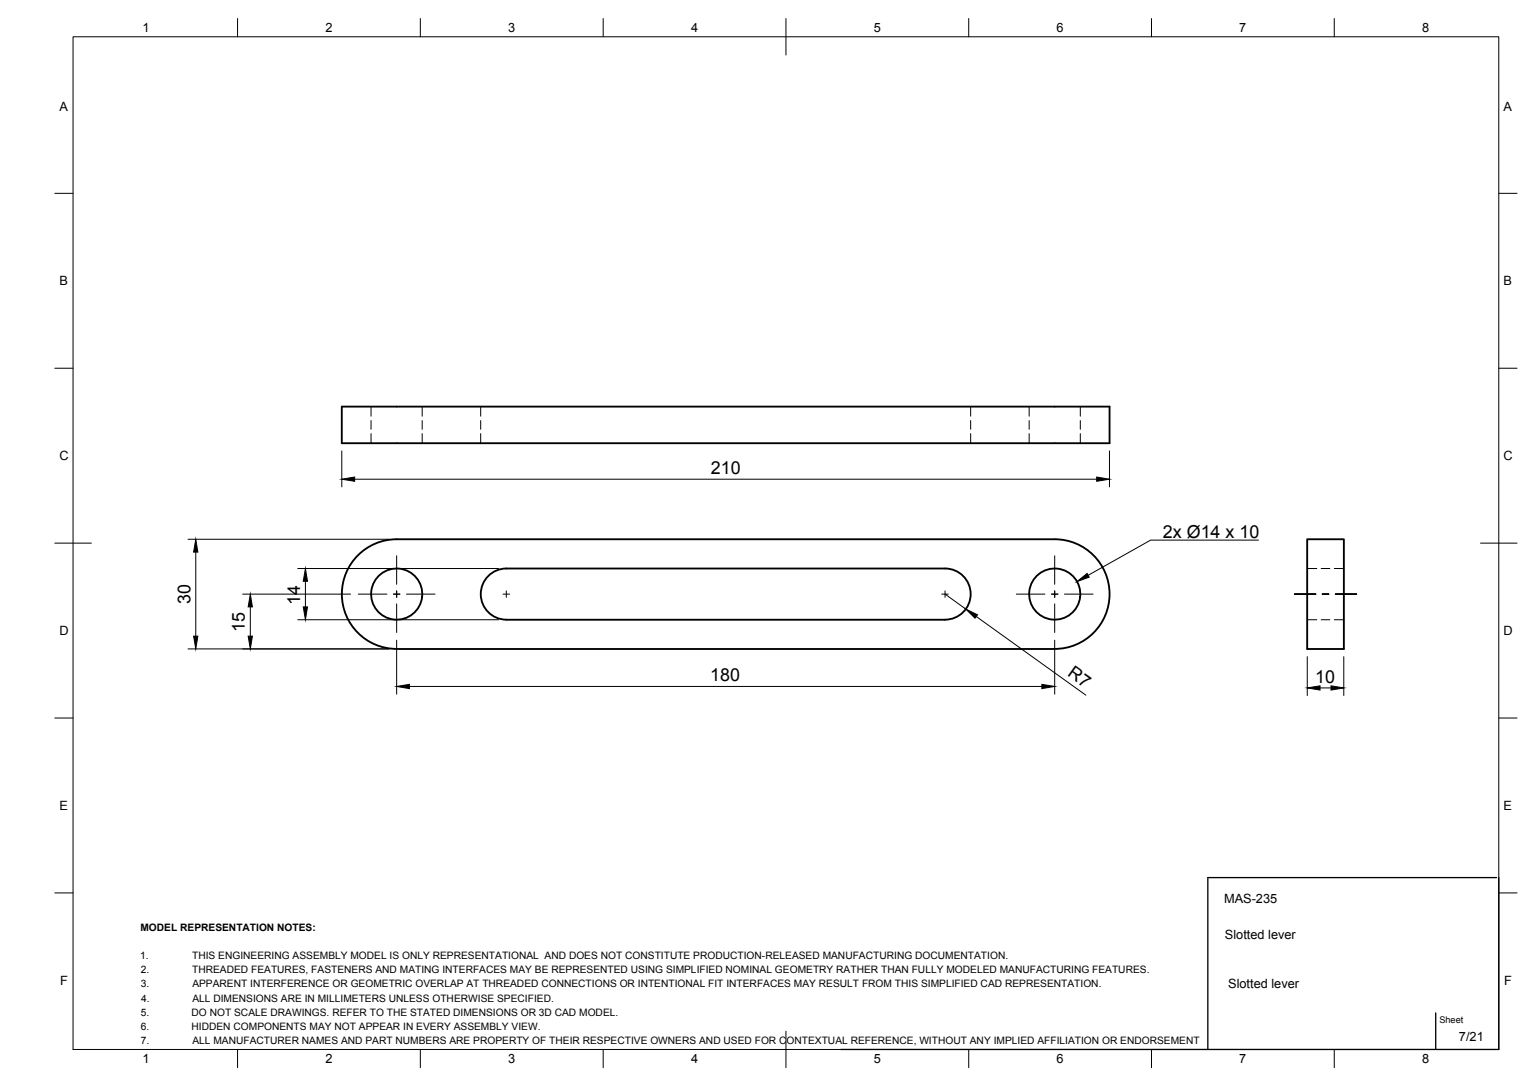
ISO-10303-21;
HEADER;
/* Generated by software containing ST-Developer
 * from STEP Tools, Inc. (www.steptools.com) 
 */

FILE_DESCRIPTION(
/* description */ ('Independent Whitworth quick-return mechanism. Crank radius40, ground-
center spacing80, lever180, connecting rod160, output guide X200. Nomi
nal stroke180 and long/short phase ratio2. Retained guide rods, replac
eable bearing sleeves and captured sliding shoe. No load or production
 rating assigned.'),
/* implementation_level */ '2;1');

FILE_NAME(
/* name */ 'Slotted lever.step',
/* time_stamp */ '2026-11-09T18:22:56-08:00',
/* author */ (''),
/* organization */ (''),
/* preprocessor_version */ 'ST-DEVELOPER v20.2',
/* originating_system */ 'Autodesk Translation Framework v15.17.0.0',
/* authorisation */ '');

FILE_SCHEMA (('AUTOMOTIVE_DESIGN { 1 0 10303 214 3 1 1 }'));
ENDSEC;

DATA;
#10=MECHANICAL_DESIGN_GEOMETRIC_PRESENTATION_REPRESENTATION('',(#223),#4388);
#183=SHAPE_REPRESENTATION_RELATIONSHIP('SRR','None',#4482,#203);
#203=ADVANCED_BREP_SHAPE_REPRESENTATION('',(#243),#4372);
#223=STYLED_ITEM('',(#4590),#243);
#243=MANIFOLD_SOLID_BREP('Body1',#2328);
#271=FACE_BOUND('',#599,.T.);
#272=FACE_BOUND('',#600,.T.);
#273=FACE_BOUND('',#601,.T.);
#274=FACE_BOUND('',#603,.T.);
#275=FACE_BOUND('',#604,.T.);
#276=FACE_BOUND('',#605,.T.);
#333=PLANE('',#2615);
#334=PLANE('',#2619);
#335=PLANE('',#2629);
#336=PLANE('',#2633);
#337=PLANE('',#2637);
#338=PLANE('',#2638);
#429=FACE_OUTER_BOUND('',#588,.T.);
#430=FACE_OUTER_BOUND('',#589,.T.);
#431=FACE_OUTER_BOUND('',#590,.T.);
#432=FACE_OUTER_BOUND('',#591,.T.);
#433=FACE_OUTER_BOUND('',#592,.T.);
#434=FACE_OUTER_BOUND('',#593,.T.);
#435=FACE_OUTER_BOUND('',#594,.T.);
#436=FACE_OUTER_BOUND('',#595,.T.);
#437=FACE_OUTER_BOUND('',#596,.T.);
#438=FACE_OUTER_BOUND('',#597,.T.);
#439=FACE_OUTER_BOUND('',#598,.T.);
#440=FACE_OUTER_BOUND('',#602,.T.);
#588=EDGE_LOOP('',(#1690,#1691,#1692,#1693));
#589=EDGE_LOOP('',(#1694,#1695,#1696,#1697));
#590=EDGE_LOOP('',(#1698,#1699,#1700,#1701));
#591=EDGE_LOOP('',(#1702,#1703,#1704,#1705));
#592=EDGE_LOOP('',(#1706,#1707,#1708,#1709));
#593=EDGE_LOOP('',(#1710,#1711,#1712,#1713));
#594=EDGE_LOOP('',(#1714,#1715,#1716,#1717));
#595=EDGE_LOOP('',(#1718,#1719,#1720,#1721));
#596=EDGE_LOOP('',(#1722,#1723,#1724,#1725));
#597=EDGE_LOOP('',(#1726,#1727,#1728,#1729));
#598=EDGE_LOOP('',(#1730,#1731,#1732,#1733));
#599=EDGE_LOOP('',(#1734,#1735,#1736,#1737));
#600=EDGE_LOOP('',(#1738));
#601=EDGE_LOOP('',(#1739));
#602=EDGE_LOOP('',(#1740,#1741,#1742,#1743));
#603=EDGE_LOOP('',(#1744,#1745,#1746,#1747));
#604=EDGE_LOOP('',(#1748));
#605=EDGE_LOOP('',(#1749));
#787=LINE('',#3813,#926);
#788=LINE('',#3815,#927);
#789=LINE('',#3817,#928);
#790=LINE('',#3818,#929);
#791=LINE('',#3823,#930);
#792=LINE('',#3827,#931);
#793=LINE('',#3829,#932);
#794=LINE('',#3830,#933);
#795=LINE('',#3838,#934);
#796=LINE('',#3844,#935);
#797=LINE('',#3849,#936);
#798=LINE('',#3851,#937);
#799=LINE('',#3853,#938);
#800=LINE('',#3854,#939);
#801=LINE('',#3860,#940);
#802=LINE('',#3863,#941);
#803=LINE('',#3865,#942);
#804=LINE('',#3866,#943);
#926=VECTOR('',#3027,10.);
#927=VECTOR('',#3028,10.);
#928=VECTOR('',#3029,10.);
#929=VECTOR('',#3030,10.);
#930=VECTOR('',#3035,10.);
#931=VECTOR('',#3040,10.);
#932=VECTOR('',#3041,10.);
#933=VECTOR('',#3042,10.);
#934=VECTOR('',#3053,7.);
#935=VECTOR('',#3060,7.);
#936=VECTOR('',#3065,10.);
#937=VECTOR('',#3066,10.);
#938=VECTOR('',#3067,10.);
#939=VECTOR('',#3068,10.);
#940=VECTOR('',#3075,10.);
#941=VECTOR('',#3078,10.);
#942=VECTOR('',#3079,10.);
#943=VECTOR('',#3080,10.);
#1057=CIRCLE('',#2617,7.);
#1058=CIRCLE('',#2618,7.);
#1059=CIRCLE('',#2621,7.);
#1060=CIRCLE('',#2622,7.);
#1061=CIRCLE('',#2624,7.);
#1062=CIRCLE('',#2625,7.);
#1063=CIRCLE('',#2627,7.);
#1064=CIRCLE('',#2628,7.);
#1065=CIRCLE('',#2631,15.);
#1066=CIRCLE('',#2632,15.);
#1067=CIRCLE('',#2635,15.);
#1068=CIRCLE('',#2636,15.);
#1191=VERTEX_POINT('',#3811);
#1192=VERTEX_POINT('',#3812);
#1193=VERTEX_POINT('',#3814);
#1194=VERTEX_POINT('',#3816);
#1195=VERTEX_POINT('',#3820);
#1196=VERTEX_POINT('',#3822);
#1197=VERTEX_POINT('',#3826);
#1198=VERTEX_POINT('',#3828);
#1199=VERTEX_POINT('',#3835);
#1200=VERTEX_POINT('',#3837);
#1201=VERTEX_POINT('',#3841);
#1202=VERTEX_POINT('',#3843);
#1203=VERTEX_POINT('',#3847);
#1204=VERTEX_POINT('',#3848);
#1205=VERTEX_POINT('',#3850);
#1206=VERTEX_POINT('',#3852);
#1207=VERTEX_POINT('',#3856);
#1208=VERTEX_POINT('',#3858);
#1209=VERTEX_POINT('',#3862);
#1210=VERTEX_POINT('',#3864);
#1381=EDGE_CURVE('',#1191,#1192,#787,.T.);
#1382=EDGE_CURVE('',#1191,#1193,#788,.T.);
#1383=EDGE_CURVE('',#1194,#1193,#789,.T.);
#1384=EDGE_CURVE('',#1192,#1194,#790,.T.);
#1385=EDGE_CURVE('',#1195,#1191,#1057,.T.);
#1386=EDGE_CURVE('',#1195,#1196,#791,.T.);
#1387=EDGE_CURVE('',#1193,#1196,#1058,.T.);
#1388=EDGE_CURVE('',#1197,#1195,#792,.T.);
#1389=EDGE_CURVE('',#1197,#1198,#793,.T.);
#1390=EDGE_CURVE('',#1196,#1198,#794,.T.);
#1391=EDGE_CURVE('',#1192,#1197,#1059,.T.);
#1392=EDGE_CURVE('',#1198,#1194,#1060,.T.);
#1393=EDGE_CURVE('',#1199,#1199,#1061,.T.);
#1394=EDGE_CURVE('',#1199,#1200,#795,.T.);
#1395=EDGE_CURVE('',#1200,#1200,#1062,.T.);
#1396=EDGE_CURVE('',#1201,#1201,#1063,.T.);
#1397=EDGE_CURVE('',#1201,#1202,#796,.T.);
#1398=EDGE_CURVE('',#1202,#1202,#1064,.T.);
#1399=EDGE_CURVE('',#1203,#1204,#797,.T.);
#1400=EDGE_CURVE('',#1204,#1205,#798,.T.);
#1401=EDGE_CURVE('',#1206,#1205,#799,.T.);
#1402=EDGE_CURVE('',#1203,#1206,#800,.T.);
#1403=EDGE_CURVE('',#1207,#1203,#1065,.T.);
#1404=EDGE_CURVE('',#1208,#1206,#1066,.T.);
#1405=EDGE_CURVE('',#1207,#1208,#801,.T.);
#1406=EDGE_CURVE('',#1209,#1207,#802,.T.);
#1407=EDGE_CURVE('',#1210,#1208,#803,.T.);
#1408=EDGE_CURVE('',#1209,#1210,#804,.T.);
#1409=EDGE_CURVE('',#1204,#1209,#1067,.T.);
#1410=EDGE_CURVE('',#1205,#1210,#1068,.T.);
#1690=ORIENTED_EDGE('',*,*,#1381,.F.);
#1691=ORIENTED_EDGE('',*,*,#1382,.T.);
#1692=ORIENTED_EDGE('',*,*,#1383,.F.);
#1693=ORIENTED_EDGE('',*,*,#1384,.F.);
#1694=ORIENTED_EDGE('',*,*,#1385,.F.);
#1695=ORIENTED_EDGE('',*,*,#1386,.T.);
#1696=ORIENTED_EDGE('',*,*,#1387,.F.);
#1697=ORIENTED_EDGE('',*,*,#1382,.F.);
#1698=ORIENTED_EDGE('',*,*,#1388,.F.);
#1699=ORIENTED_EDGE('',*,*,#1389,.T.);
#1700=ORIENTED_EDGE('',*,*,#1390,.F.);
#1701=ORIENTED_EDGE('',*,*,#1386,.F.);
#1702=ORIENTED_EDGE('',*,*,#1391,.F.);
#1703=ORIENTED_EDGE('',*,*,#1384,.T.);
#1704=ORIENTED_EDGE('',*,*,#1392,.F.);
#1705=ORIENTED_EDGE('',*,*,#1389,.F.);
#1706=ORIENTED_EDGE('',*,*,#1393,.F.);
#1707=ORIENTED_EDGE('',*,*,#1394,.T.);
#1708=ORIENTED_EDGE('',*,*,#1395,.F.);
#1709=ORIENTED_EDGE('',*,*,#1394,.F.);
#1710=ORIENTED_EDGE('',*,*,#1396,.F.);
#1711=ORIENTED_EDGE('',*,*,#1397,.T.);
#1712=ORIENTED_EDGE('',*,*,#1398,.F.);
#1713=ORIENTED_EDGE('',*,*,#1397,.F.);
#1714=ORIENTED_EDGE('',*,*,#1399,.T.);
#1715=ORIENTED_EDGE('',*,*,#1400,.T.);
#1716=ORIENTED_EDGE('',*,*,#1401,.F.);
#1717=ORIENTED_EDGE('',*,*,#1402,.F.);
#1718=ORIENTED_EDGE('',*,*,#1403,.T.);
#1719=ORIENTED_EDGE('',*,*,#1402,.T.);
#1720=ORIENTED_EDGE('',*,*,#1404,.F.);
#1721=ORIENTED_EDGE('',*,*,#1405,.F.);
#1722=ORIENTED_EDGE('',*,*,#1406,.T.);
#1723=ORIENTED_EDGE('',*,*,#1405,.T.);
#1724=ORIENTED_EDGE('',*,*,#1407,.F.);
#1725=ORIENTED_EDGE('',*,*,#1408,.F.);
#1726=ORIENTED_EDGE('',*,*,#1409,.T.);
#1727=ORIENTED_EDGE('',*,*,#1408,.T.);
#1728=ORIENTED_EDGE('',*,*,#1410,.F.);
#1729=ORIENTED_EDGE('',*,*,#1400,.F.);
#1730=ORIENTED_EDGE('',*,*,#1410,.T.);
#1731=ORIENTED_EDGE('',*,*,#1407,.T.);
#1732=ORIENTED_EDGE('',*,*,#1404,.T.);
#1733=ORIENTED_EDGE('',*,*,#1401,.T.);
#1734=ORIENTED_EDGE('',*,*,#1381,.T.);
#1735=ORIENTED_EDGE('',*,*,#1391,.T.);
#1736=ORIENTED_EDGE('',*,*,#1388,.T.);
#1737=ORIENTED_EDGE('',*,*,#1385,.T.);
#1738=ORIENTED_EDGE('',*,*,#1393,.T.);
#1739=ORIENTED_EDGE('',*,*,#1396,.T.);
#1740=ORIENTED_EDGE('',*,*,#1409,.F.);
#1741=ORIENTED_EDGE('',*,*,#1399,.F.);
#1742=ORIENTED_EDGE('',*,*,#1403,.F.);
#1743=ORIENTED_EDGE('',*,*,#1406,.F.);
#1744=ORIENTED_EDGE('',*,*,#1383,.T.);
#1745=ORIENTED_EDGE('',*,*,#1387,.T.);
#1746=ORIENTED_EDGE('',*,*,#1390,.T.);
#1747=ORIENTED_EDGE('',*,*,#1392,.T.);
#1748=ORIENTED_EDGE('',*,*,#1395,.T.);
#1749=ORIENTED_EDGE('',*,*,#1398,.T.);
#2126=CYLINDRICAL_SURFACE('',#2616,7.);
#2127=CYLINDRICAL_SURFACE('',#2620,7.);
#2128=CYLINDRICAL_SURFACE('',#2623,7.);
#2129=CYLINDRICAL_SURFACE('',#2626,7.);
#2130=CYLINDRICAL_SURFACE('',#2630,15.);
#2131=CYLINDRICAL_SURFACE('',#2634,15.);
#2201=ADVANCED_FACE('',(#429),#333,.F.);
#2202=ADVANCED_FACE('',(#430),#2126,.F.);
#2203=ADVANCED_FACE('',(#431),#334,.F.);
#2204=ADVANCED_FACE('',(#432),#2127,.F.);
#2205=ADVANCED_FACE('',(#433),#2128,.F.);
#2206=ADVANCED_FACE('',(#434),#2129,.F.);
#2207=ADVANCED_FACE('',(#435),#335,.T.);
#2208=ADVANCED_FACE('',(#436),#2130,.T.);
#2209=ADVANCED_FACE('',(#437),#336,.T.);
#2210=ADVANCED_FACE('',(#438),#2131,.T.);
#2211=ADVANCED_FACE('',(#439,#271,#272,#273),#337,.T.);
#2212=ADVANCED_FACE('',(#440,#274,#275,#276),#338,.F.);
#2328=CLOSED_SHELL('',(#2201,#2202,#2203,#2204,#2205,#2206,#2207,#2208,
#2209,#2210,#2211,#2212));
#2614=AXIS2_PLACEMENT_3D('',#3809,#3023,#3024);
#2615=AXIS2_PLACEMENT_3D('',#3810,#3025,#3026);
#2616=AXIS2_PLACEMENT_3D('',#3819,#3031,#3032);
#2617=AXIS2_PLACEMENT_3D('',#3821,#3033,#3034);
#2618=AXIS2_PLACEMENT_3D('',#3824,#3036,#3037);
#2619=AXIS2_PLACEMENT_3D('',#3825,#3038,#3039);
#2620=AXIS2_PLACEMENT_3D('',#3831,#3043,#3044);
#2621=AXIS2_PLACEMENT_3D('',#3832,#3045,#3046);
#2622=AXIS2_PLACEMENT_3D('',#3833,#3047,#3048);
#2623=AXIS2_PLACEMENT_3D('',#3834,#3049,#3050);
#2624=AXIS2_PLACEMENT_3D('',#3836,#3051,#3052);
#2625=AXIS2_PLACEMENT_3D('',#3839,#3054,#3055);
#2626=AXIS2_PLACEMENT_3D('',#3840,#3056,#3057);
#2627=AXIS2_PLACEMENT_3D('',#3842,#3058,#3059);
#2628=AXIS2_PLACEMENT_3D('',#3845,#3061,#3062);
#2629=AXIS2_PLACEMENT_3D('',#3846,#3063,#3064);
#2630=AXIS2_PLACEMENT_3D('',#3855,#3069,#3070);
#2631=AXIS2_PLACEMENT_3D('',#3857,#3071,#3072);
#2632=AXIS2_PLACEMENT_3D('',#3859,#3073,#3074);
#2633=AXIS2_PLACEMENT_3D('',#3861,#3076,#3077);
#2634=AXIS2_PLACEMENT_3D('',#3867,#3081,#3082);
#2635=AXIS2_PLACEMENT_3D('',#3868,#3083,#3084);
#2636=AXIS2_PLACEMENT_3D('',#3869,#3085,#3086);
#2637=AXIS2_PLACEMENT_3D('',#3870,#3087,#3088);
#2638=AXIS2_PLACEMENT_3D('',#3871,#3089,#3090);
#3023=DIRECTION('axis',(0.,0.,1.));
#3024=DIRECTION('refdir',(1.,0.,0.));
#3025=DIRECTION('center_axis',(0.,-1.,0.));
#3026=DIRECTION('ref_axis',(-1.,0.,0.));
#3027=DIRECTION('',(-1.,0.,0.));
#3028=DIRECTION('',(0.,0.,-1.));
#3029=DIRECTION('',(1.,0.,0.));
#3030=DIRECTION('',(0.,0.,-1.));
#3031=DIRECTION('center_axis',(0.,0.,-1.));
#3032=DIRECTION('ref_axis',(0.,-1.,0.));
#3033=DIRECTION('center_axis',(0.,0.,-1.));
#3034=DIRECTION('ref_axis',(0.,-1.,0.));
#3035=DIRECTION('',(0.,0.,-1.));
#3036=DIRECTION('center_axis',(0.,0.,1.));
#3037=DIRECTION('ref_axis',(0.,-1.,0.));
#3038=DIRECTION('center_axis',(0.,1.,0.));
#3039=DIRECTION('ref_axis',(1.,0.,0.));
#3040=DIRECTION('',(1.,0.,0.));
#3041=DIRECTION('',(0.,0.,-1.));
#3042=DIRECTION('',(-1.,0.,0.));
#3043=DIRECTION('center_axis',(0.,0.,-1.));
#3044=DIRECTION('ref_axis',(0.,1.,0.));
#3045=DIRECTION('center_axis',(0.,0.,-1.));
#3046=DIRECTION('ref_axis',(0.,1.,0.));
#3047=DIRECTION('center_axis',(0.,0.,1.));
#3048=DIRECTION('ref_axis',(0.,1.,0.));
#3049=DIRECTION('center_axis',(0.,0.,-1.));
#3050=DIRECTION('ref_axis',(1.,0.,0.));
#3051=DIRECTION('center_axis',(0.,0.,-1.));
#3052=DIRECTION('ref_axis',(1.,0.,0.));
#3053=DIRECTION('',(0.,0.,-1.));
#3054=DIRECTION('center_axis',(0.,0.,1.));
#3055=DIRECTION('ref_axis',(1.,0.,0.));
#3056=DIRECTION('center_axis',(0.,0.,-1.));
#3057=DIRECTION('ref_axis',(1.,0.,0.));
#3058=DIRECTION('center_axis',(0.,0.,-1.));
#3059=DIRECTION('ref_axis',(1.,0.,0.));
#3060=DIRECTION('',(0.,0.,-1.));
#3061=DIRECTION('center_axis',(0.,0.,1.));
#3062=DIRECTION('ref_axis',(1.,0.,0.));
#3063=DIRECTION('center_axis',(0.,1.,0.));
#3064=DIRECTION('ref_axis',(-1.,0.,0.));
#3065=DIRECTION('',(-1.,0.,0.));
#3066=DIRECTION('',(0.,0.,1.));
#3067=DIRECTION('',(-1.,0.,0.));
#3068=DIRECTION('',(0.,0.,1.));
#3069=DIRECTION('center_axis',(0.,0.,1.));
#3070=DIRECTION('ref_axis',(0.,-1.,0.));
#3071=DIRECTION('center_axis',(0.,0.,1.));
#3072=DIRECTION('ref_axis',(0.,-1.,0.));
#3073=DIRECTION('center_axis',(0.,0.,1.));
#3074=DIRECTION('ref_axis',(0.,-1.,0.));
#3075=DIRECTION('',(0.,0.,1.));
#3076=DIRECTION('center_axis',(0.,-1.,0.));
#3077=DIRECTION('ref_axis',(1.,0.,0.));
#3078=DIRECTION('',(1.,0.,0.));
#3079=DIRECTION('',(1.,0.,0.));
#3080=DIRECTION('',(0.,0.,1.));
#3081=DIRECTION('center_axis',(0.,0.,1.));
#3082=DIRECTION('ref_axis',(0.,1.,0.));
#3083=DIRECTION('center_axis',(0.,0.,1.));
#3084=DIRECTION('ref_axis',(0.,1.,0.));
#3085=DIRECTION('center_axis',(0.,0.,1.));
#3086=DIRECTION('ref_axis',(0.,1.,0.));
#3087=DIRECTION('center_axis',(0.,0.,1.));
#3088=DIRECTION('ref_axis',(1.,0.,0.));
#3089=DIRECTION('center_axis',(0.,0.,1.));
#3090=DIRECTION('ref_axis',(1.,0.,0.));
#3809=CARTESIAN_POINT('',(0.,0.,0.));
#3810=CARTESIAN_POINT('Origin',(150.,-7.,10.));
#3811=CARTESIAN_POINT('',(150.,-7.,10.));
#3812=CARTESIAN_POINT('',(30.,-7.,10.));
#3813=CARTESIAN_POINT('',(120.,-7.,10.));
#3814=CARTESIAN_POINT('',(150.,-7.,0.));
#3815=CARTESIAN_POINT('',(150.,-7.,10.));
#3816=CARTESIAN_POINT('',(30.,-7.,0.));
#3817=CARTESIAN_POINT('',(120.,-7.,0.));
#3818=CARTESIAN_POINT('',(30.,-7.,10.));
#3819=CARTESIAN_POINT('Origin',(150.,0.,10.));
#3820=CARTESIAN_POINT('',(150.,7.,10.));
#3821=CARTESIAN_POINT('Origin',(150.,0.,10.));
#3822=CARTESIAN_POINT('',(150.,7.,0.));
#3823=CARTESIAN_POINT('',(150.,7.,10.));
#3824=CARTESIAN_POINT('Origin',(150.,0.,0.));
#3825=CARTESIAN_POINT('Origin',(30.,7.,10.));
#3826=CARTESIAN_POINT('',(30.,7.,10.));
#3827=CARTESIAN_POINT('',(60.,7.,10.));
#3828=CARTESIAN_POINT('',(30.,7.,0.));
#3829=CARTESIAN_POINT('',(30.,7.,10.));
#3830=CARTESIAN_POINT('',(60.,7.,0.));
#3831=CARTESIAN_POINT('Origin',(30.,0.,10.));
#3832=CARTESIAN_POINT('Origin',(30.,0.,10.));
#3833=CARTESIAN_POINT('Origin',(30.,0.,0.));
#3834=CARTESIAN_POINT('Origin',(0.,0.,5.));
#3835=CARTESIAN_POINT('',(-7.,8.57252759403147E-16,10.));
#3836=CARTESIAN_POINT('Origin',(0.,0.,10.));
#3837=CARTESIAN_POINT('',(-7.,8.57252759403147E-16,0.));
#3838=CARTESIAN_POINT('',(-7.,8.57252759403147E-16,5.));
#3839=CARTESIAN_POINT('Origin',(0.,0.,0.));
#3840=CARTESIAN_POINT('Origin',(180.,0.,5.));
#3841=CARTESIAN_POINT('',(173.,8.57252759403147E-16,10.));
#3842=CARTESIAN_POINT('Origin',(180.,0.,10.));
#3843=CARTESIAN_POINT('',(173.,8.57252759403147E-16,0.));
#3844=CARTESIAN_POINT('',(173.,8.57252759403147E-16,5.));
#3845=CARTESIAN_POINT('Origin',(180.,0.,0.));
#3846=CARTESIAN_POINT('Origin',(180.,15.,0.));
#3847=CARTESIAN_POINT('',(180.,15.,0.));
#3848=CARTESIAN_POINT('',(0.,15.,0.));
#3849=CARTESIAN_POINT('',(180.,15.,0.));
#3850=CARTESIAN_POINT('',(0.,15.,10.));
#3851=CARTESIAN_POINT('',(0.,15.,0.));
#3852=CARTESIAN_POINT('',(180.,15.,10.));
#3853=CARTESIAN_POINT('',(180.,15.,10.));
#3854=CARTESIAN_POINT('',(180.,15.,0.));
#3855=CARTESIAN_POINT('Origin',(180.,0.,0.));
#3856=CARTESIAN_POINT('',(180.,-15.,0.));
#3857=CARTESIAN_POINT('Origin',(180.,0.,0.));
#3858=CARTESIAN_POINT('',(180.,-15.,10.));
#3859=CARTESIAN_POINT('Origin',(180.,0.,10.));
#3860=CARTESIAN_POINT('',(180.,-15.,0.));
#3861=CARTESIAN_POINT('Origin',(0.,-15.,0.));
#3862=CARTESIAN_POINT('',(-1.83697019872103E-15,-15.,0.));
#3863=CARTESIAN_POINT('',(0.,-15.,0.));
#3864=CARTESIAN_POINT('',(-1.83697019872103E-15,-15.,10.));
#3865=CARTESIAN_POINT('',(0.,-15.,10.));
#3866=CARTESIAN_POINT('',(-1.83697019872103E-15,-15.,0.));
#3867=CARTESIAN_POINT('Origin',(0.,0.,0.));
#3868=CARTESIAN_POINT('Origin',(0.,0.,0.));
#3869=CARTESIAN_POINT('Origin',(0.,0.,10.));
#3870=CARTESIAN_POINT('Origin',(90.,0.,10.));
#3871=CARTESIAN_POINT('Origin',(90.,0.,0.));
#4350=UNCERTAINTY_MEASURE_WITH_UNIT(LENGTH_MEASURE(0.01),#4389,
'DISTANCE_ACCURACY_VALUE',
'Maximum model space distance between geometric entities at asserted c
onnectivities');
#4366=UNCERTAINTY_MEASURE_WITH_UNIT(LENGTH_MEASURE(0.01),#4389,
'DISTANCE_ACCURACY_VALUE',
'Maximum model space distance between geometric entities at asserted c
onnectivities');
#4372=(
GEOMETRIC_REPRESENTATION_CONTEXT(3)
GLOBAL_UNCERTAINTY_ASSIGNED_CONTEXT((#4350))
GLOBAL_UNIT_ASSIGNED_CONTEXT((#4389,#4391,#4392))
REPRESENTATION_CONTEXT('','3D')
);
#4388=(
GEOMETRIC_REPRESENTATION_CONTEXT(3)
GLOBAL_UNCERTAINTY_ASSIGNED_CONTEXT((#4366))
GLOBAL_UNIT_ASSIGNED_CONTEXT((#4389,#4391,#4392))
REPRESENTATION_CONTEXT('','3D')
);
#4389=(
LENGTH_UNIT()
NAMED_UNIT(*)
SI_UNIT(.MILLI.,.METRE.)
);
#4391=(
NAMED_UNIT(*)
PLANE_ANGLE_UNIT()
SI_UNIT($,.RADIAN.)
);
#4392=(
NAMED_UNIT(*)
SI_UNIT($,.STERADIAN.)
SOLID_ANGLE_UNIT()
);
#4398=SHAPE_DEFINITION_REPRESENTATION(#4419,#4482);
#4419=PRODUCT_DEFINITION_SHAPE('',$,#4504);
#4482=SHAPE_REPRESENTATION('',(#2614),#4372);
#4498=PRODUCT_DEFINITION_CONTEXT('part definition',#4563,'design');
#4504=PRODUCT_DEFINITION('Slotted lever','Slotted lever',#4525,#4498);
#4525=PRODUCT_DEFINITION_FORMATION('',$,#4570);
#4563=APPLICATION_CONTEXT(
'Core Data for Automotive Mechanical Design Process');
#4564=PRODUCT_CONTEXT('part definition',#4563,'mechanical');
#4570=PRODUCT('Slotted lever','Slotted lever','Slotted lever',(#4564));
#4590=PRESENTATION_STYLE_ASSIGNMENT((#4604));
#4604=SURFACE_STYLE_USAGE(.BOTH.,#4618);
#4618=SURFACE_SIDE_STYLE('',(#4632));
#4632=SURFACE_STYLE_FILL_AREA(#4646);
#4646=FILL_AREA_STYLE('Sky blue',(#4660));
#4660=FILL_AREA_STYLE_COLOUR('Sky blue',#4674);
#4674=COLOUR_RGB('Sky blue',0.317647058823529,0.686274509803922,0.890196078431372);
ENDSEC;
END-ISO-10303-21;
